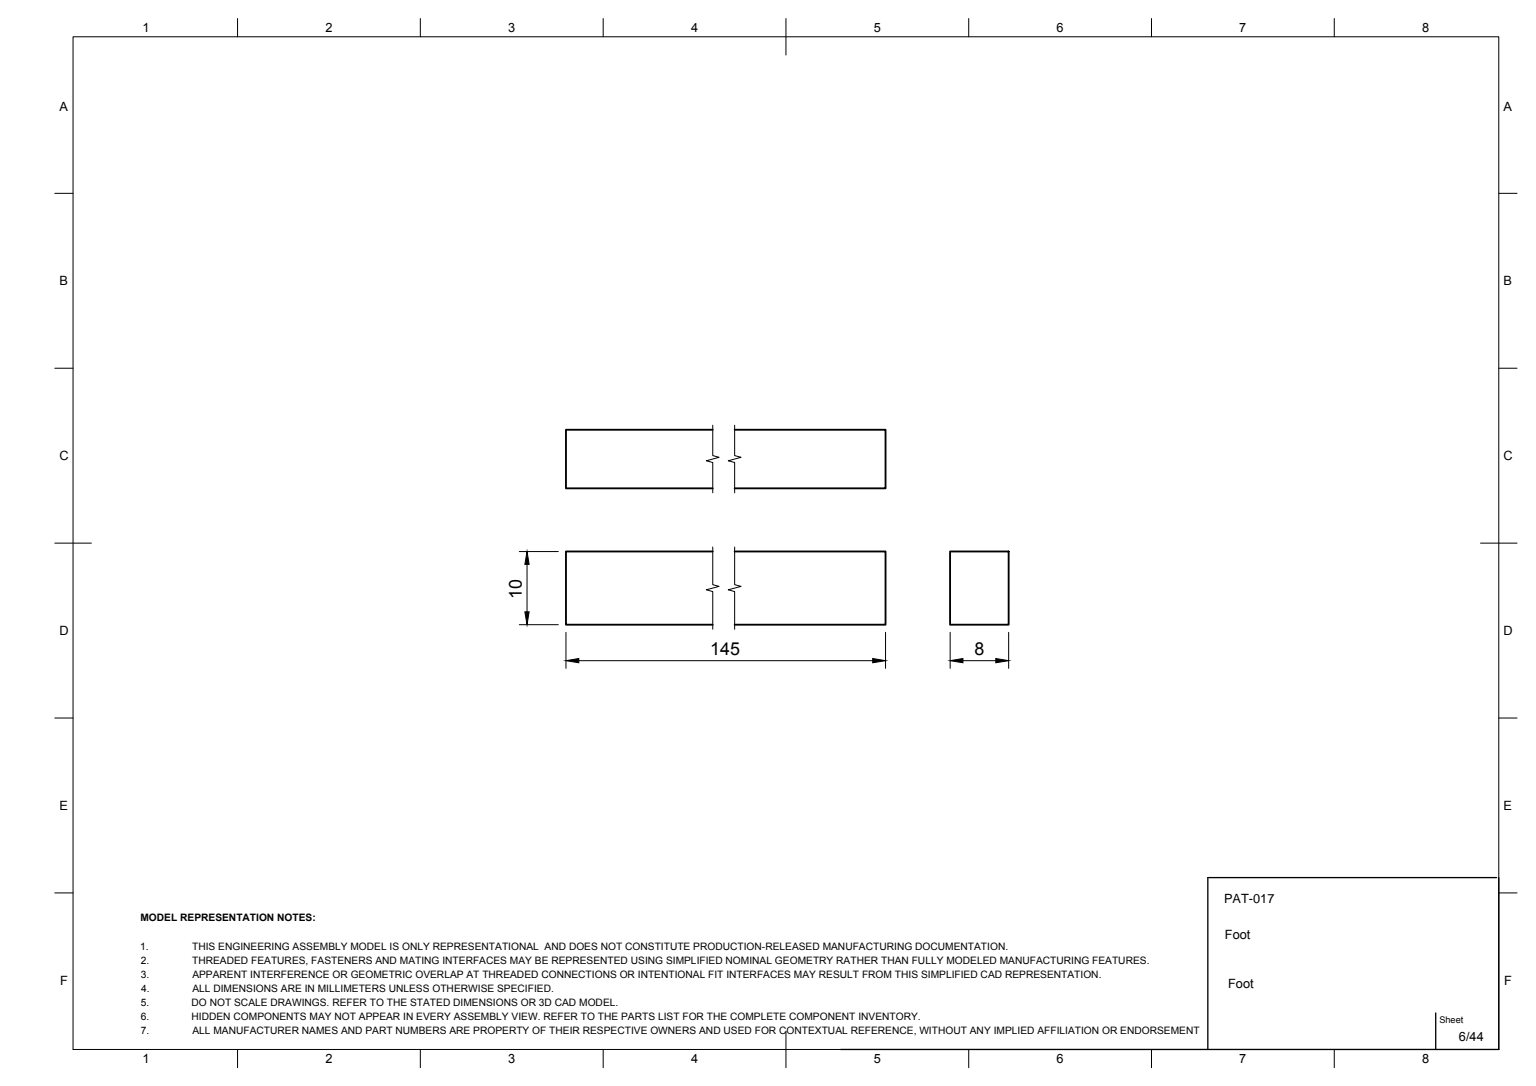
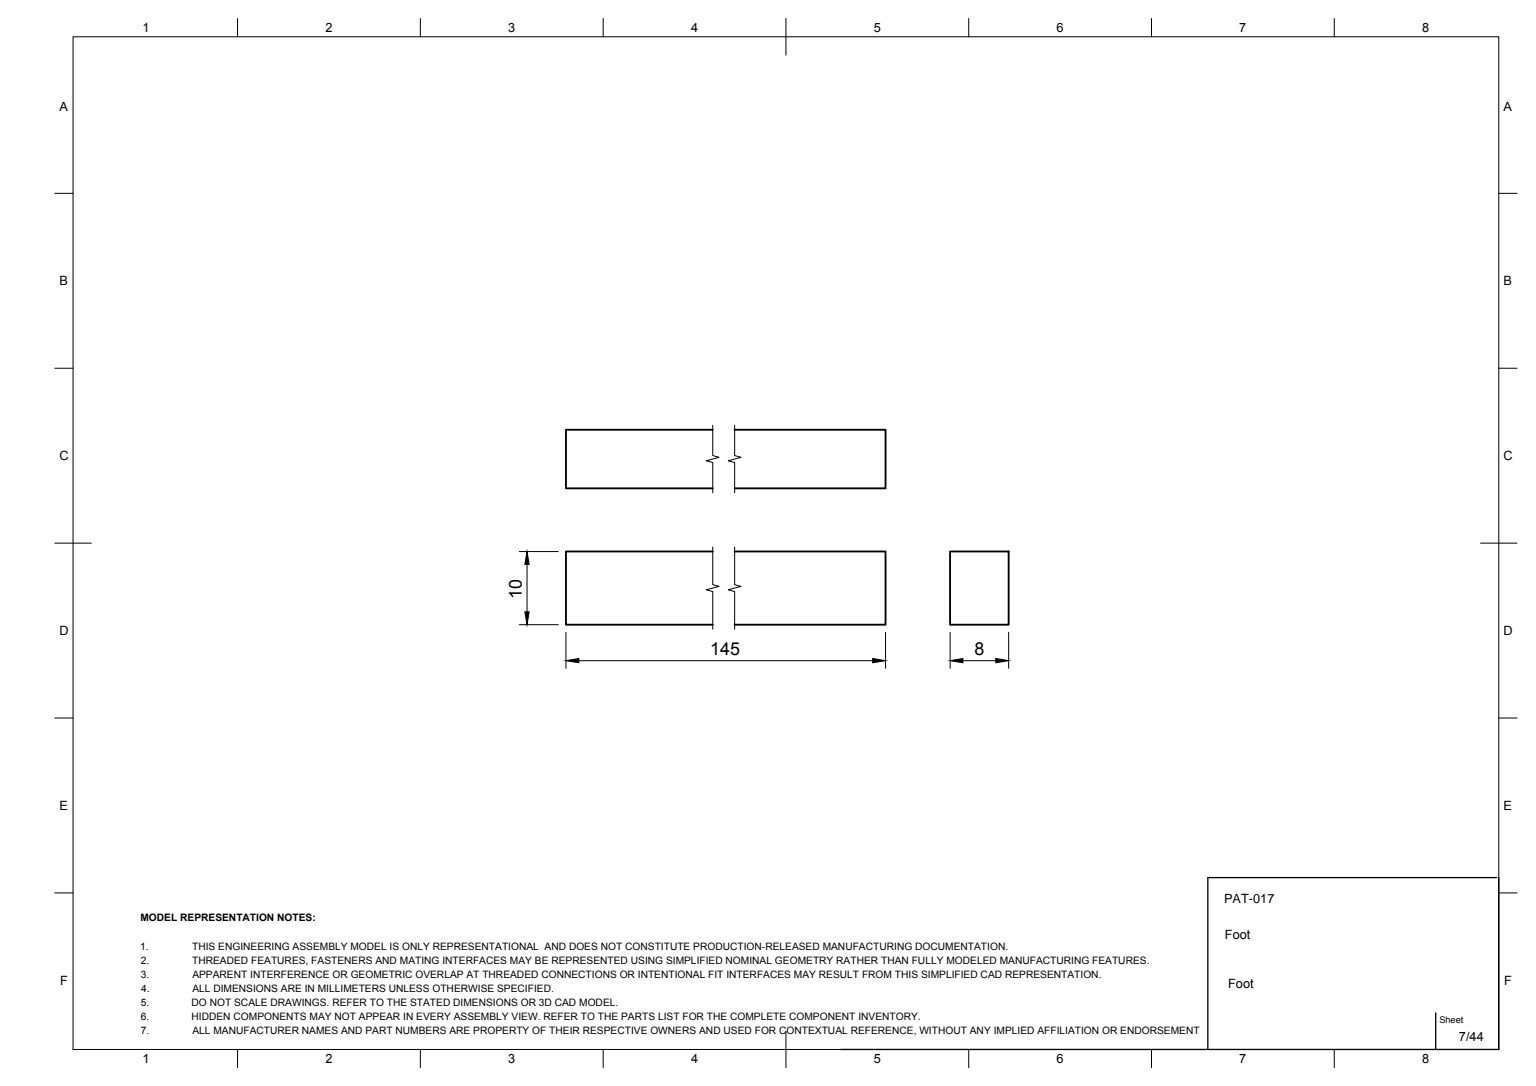
ISO-10303-21;
HEADER;
/* Generated by software containing ST-Developer
 * from STEP Tools, Inc. (www.steptools.com) 
 */

FILE_DESCRIPTION(
/* description */ ('Cam-and-follower valve demonstrator'),
/* implementation_level */ '2;1');

FILE_NAME(
/* name */ 'Foot.step',
/* time_stamp */ '2026-10-28T03:25:17-07:00',
/* author */ (''),
/* organization */ (''),
/* preprocessor_version */ 'ST-DEVELOPER v20.2',
/* originating_system */ 'Autodesk Translation Framework v15.17.0.0',
/* authorisation */ '');

FILE_SCHEMA (('AUTOMOTIVE_DESIGN { 1 0 10303 214 3 1 1 }'));
ENDSEC;

DATA;
#10=MECHANICAL_DESIGN_GEOMETRIC_PRESENTATION_REPRESENTATION('',(#413),#12896);
#341=SHAPE_REPRESENTATION_RELATIONSHIP('SRR','None',#13057,#377);
#377=ADVANCED_BREP_SHAPE_REPRESENTATION('',(#456),#12857);
#413=STYLED_ITEM('',(#13344),#456);
#456=MANIFOLD_SOLID_BREP('Body1',#6180);
#1112=FACE_OUTER_BOUND('',#1493,.T.);
#1113=FACE_OUTER_BOUND('',#1494,.T.);
#1114=FACE_OUTER_BOUND('',#1495,.T.);
#1115=FACE_OUTER_BOUND('',#1496,.T.);
#1116=FACE_OUTER_BOUND('',#1497,.T.);
#1117=FACE_OUTER_BOUND('',#1498,.T.);
#1493=EDGE_LOOP('',(#4179,#4180,#4181,#4182));
#1494=EDGE_LOOP('',(#4183,#4184,#4185,#4186));
#1495=EDGE_LOOP('',(#4187,#4188,#4189,#4190));
#1496=EDGE_LOOP('',(#4191,#4192,#4193,#4194));
#1497=EDGE_LOOP('',(#4195,#4196,#4197,#4198));
#1498=EDGE_LOOP('',(#4199,#4200,#4201,#4202));
#2025=LINE('',#9514,#2447);
#2026=LINE('',#9516,#2448);
#2027=LINE('',#9518,#2449);
#2028=LINE('',#9519,#2450);
#2029=LINE('',#9522,#2451);
#2030=LINE('',#9524,#2452);
#2031=LINE('',#9525,#2453);
#2032=LINE('',#9528,#2454);
#2033=LINE('',#9530,#2455);
#2034=LINE('',#9531,#2456);
#2035=LINE('',#9533,#2457);
#2036=LINE('',#9534,#2458);
#2447=VECTOR('',#7512,1.);
#2448=VECTOR('',#7513,1.);
#2449=VECTOR('',#7514,1.);
#2450=VECTOR('',#7515,1.);
#2451=VECTOR('',#7518,1.);
#2452=VECTOR('',#7519,1.);
#2453=VECTOR('',#7520,1.);
#2454=VECTOR('',#7523,1.);
#2455=VECTOR('',#7524,1.);
#2456=VECTOR('',#7525,1.);
#2457=VECTOR('',#7528,1.);
#2458=VECTOR('',#7529,1.);
#2867=VERTEX_POINT('',#9512);
#2868=VERTEX_POINT('',#9513);
#2869=VERTEX_POINT('',#9515);
#2870=VERTEX_POINT('',#9517);
#2871=VERTEX_POINT('',#9521);
#2872=VERTEX_POINT('',#9523);
#2873=VERTEX_POINT('',#9527);
#2874=VERTEX_POINT('',#9529);
#3386=EDGE_CURVE('',#2867,#2868,#2025,.T.);
#3387=EDGE_CURVE('',#2868,#2869,#2026,.T.);
#3388=EDGE_CURVE('',#2870,#2869,#2027,.T.);
#3389=EDGE_CURVE('',#2867,#2870,#2028,.T.);
#3390=EDGE_CURVE('',#2871,#2867,#2029,.T.);
#3391=EDGE_CURVE('',#2872,#2870,#2030,.T.);
#3392=EDGE_CURVE('',#2871,#2872,#2031,.T.);
#3393=EDGE_CURVE('',#2873,#2871,#2032,.T.);
#3394=EDGE_CURVE('',#2874,#2872,#2033,.T.);
#3395=EDGE_CURVE('',#2873,#2874,#2034,.T.);
#3396=EDGE_CURVE('',#2868,#2873,#2035,.T.);
#3397=EDGE_CURVE('',#2869,#2874,#2036,.T.);
#4179=ORIENTED_EDGE('',*,*,#3386,.T.);
#4180=ORIENTED_EDGE('',*,*,#3387,.T.);
#4181=ORIENTED_EDGE('',*,*,#3388,.F.);
#4182=ORIENTED_EDGE('',*,*,#3389,.F.);
#4183=ORIENTED_EDGE('',*,*,#3390,.T.);
#4184=ORIENTED_EDGE('',*,*,#3389,.T.);
#4185=ORIENTED_EDGE('',*,*,#3391,.F.);
#4186=ORIENTED_EDGE('',*,*,#3392,.F.);
#4187=ORIENTED_EDGE('',*,*,#3393,.T.);
#4188=ORIENTED_EDGE('',*,*,#3392,.T.);
#4189=ORIENTED_EDGE('',*,*,#3394,.F.);
#4190=ORIENTED_EDGE('',*,*,#3395,.F.);
#4191=ORIENTED_EDGE('',*,*,#3396,.T.);
#4192=ORIENTED_EDGE('',*,*,#3395,.T.);
#4193=ORIENTED_EDGE('',*,*,#3397,.F.);
#4194=ORIENTED_EDGE('',*,*,#3387,.F.);
#4195=ORIENTED_EDGE('',*,*,#3397,.T.);
#4196=ORIENTED_EDGE('',*,*,#3394,.T.);
#4197=ORIENTED_EDGE('',*,*,#3391,.T.);
#4198=ORIENTED_EDGE('',*,*,#3388,.T.);
#4199=ORIENTED_EDGE('',*,*,#3396,.F.);
#4200=ORIENTED_EDGE('',*,*,#3386,.F.);
#4201=ORIENTED_EDGE('',*,*,#3390,.F.);
#4202=ORIENTED_EDGE('',*,*,#3393,.F.);
#5608=PLANE('',#6655);
#5609=PLANE('',#6656);
#5610=PLANE('',#6657);
#5611=PLANE('',#6658);
#5612=PLANE('',#6659);
#5613=PLANE('',#6660);
#5828=ADVANCED_FACE('',(#1112),#5608,.T.);
#5829=ADVANCED_FACE('',(#1113),#5609,.T.);
#5830=ADVANCED_FACE('',(#1114),#5610,.T.);
#5831=ADVANCED_FACE('',(#1115),#5611,.T.);
#5832=ADVANCED_FACE('',(#1116),#5612,.T.);
#5833=ADVANCED_FACE('',(#1117),#5613,.F.);
#6180=CLOSED_SHELL('',(#5828,#5829,#5830,#5831,#5832,#5833));
#6654=AXIS2_PLACEMENT_3D('',#9510,#7508,#7509);
#6655=AXIS2_PLACEMENT_3D('',#9511,#7510,#7511);
#6656=AXIS2_PLACEMENT_3D('',#9520,#7516,#7517);
#6657=AXIS2_PLACEMENT_3D('',#9526,#7521,#7522);
#6658=AXIS2_PLACEMENT_3D('',#9532,#7526,#7527);
#6659=AXIS2_PLACEMENT_3D('',#9535,#7530,#7531);
#6660=AXIS2_PLACEMENT_3D('',#9536,#7532,#7533);
#7508=DIRECTION('axis',(0.,0.,1.));
#7509=DIRECTION('refdir',(1.,0.,0.));
#7510=DIRECTION('center_axis',(0.,1.,0.));
#7511=DIRECTION('ref_axis',(-1.,0.,0.));
#7512=DIRECTION('',(-1.,0.,0.));
#7513=DIRECTION('',(0.,0.,1.));
#7514=DIRECTION('',(-1.,0.,0.));
#7515=DIRECTION('',(0.,0.,1.));
#7516=DIRECTION('center_axis',(1.,0.,0.));
#7517=DIRECTION('ref_axis',(0.,1.,0.));
#7518=DIRECTION('',(0.,1.,0.));
#7519=DIRECTION('',(0.,1.,0.));
#7520=DIRECTION('',(0.,0.,1.));
#7521=DIRECTION('center_axis',(0.,-1.,0.));
#7522=DIRECTION('ref_axis',(1.,0.,0.));
#7523=DIRECTION('',(1.,0.,0.));
#7524=DIRECTION('',(1.,0.,0.));
#7525=DIRECTION('',(0.,0.,1.));
#7526=DIRECTION('center_axis',(-1.,0.,0.));
#7527=DIRECTION('ref_axis',(0.,-1.,0.));
#7528=DIRECTION('',(0.,-1.,0.));
#7529=DIRECTION('',(0.,-1.,0.));
#7530=DIRECTION('center_axis',(0.,0.,1.));
#7531=DIRECTION('ref_axis',(1.,0.,0.));
#7532=DIRECTION('center_axis',(0.,0.,1.));
#7533=DIRECTION('ref_axis',(1.,0.,0.));
#9510=CARTESIAN_POINT('',(0.,0.,0.));
#9511=CARTESIAN_POINT('Origin',(-5.,9.,-0.8));
#9512=CARTESIAN_POINT('',(-5.,9.,-0.8));
#9513=CARTESIAN_POINT('',(-6.,9.,-0.8));
#9514=CARTESIAN_POINT('',(-5.,9.,-0.8));
#9515=CARTESIAN_POINT('',(-6.,9.,0.));
#9516=CARTESIAN_POINT('',(-6.,9.,-0.8));
#9517=CARTESIAN_POINT('',(-5.,9.,0.));
#9518=CARTESIAN_POINT('',(-5.,9.,0.));
#9519=CARTESIAN_POINT('',(-5.,9.,-0.8));
#9520=CARTESIAN_POINT('Origin',(-5.,-5.5,-0.8));
#9521=CARTESIAN_POINT('',(-5.,-5.5,-0.8));
#9522=CARTESIAN_POINT('',(-5.,-5.5,-0.8));
#9523=CARTESIAN_POINT('',(-5.,-5.5,0.));
#9524=CARTESIAN_POINT('',(-5.,-5.5,0.));
#9525=CARTESIAN_POINT('',(-5.,-5.5,-0.8));
#9526=CARTESIAN_POINT('Origin',(-6.,-5.5,-0.8));
#9527=CARTESIAN_POINT('',(-6.,-5.5,-0.8));
#9528=CARTESIAN_POINT('',(-6.,-5.5,-0.8));
#9529=CARTESIAN_POINT('',(-6.,-5.5,0.));
#9530=CARTESIAN_POINT('',(-6.,-5.5,0.));
#9531=CARTESIAN_POINT('',(-6.,-5.5,-0.8));
#9532=CARTESIAN_POINT('Origin',(-6.,9.,-0.8));
#9533=CARTESIAN_POINT('',(-6.,9.,-0.8));
#9534=CARTESIAN_POINT('',(-6.,9.,0.));
#9535=CARTESIAN_POINT('Origin',(-5.5,1.75,0.));
#9536=CARTESIAN_POINT('Origin',(-5.5,1.75,-0.8));
#12814=UNCERTAINTY_MEASURE_WITH_UNIT(LENGTH_MEASURE(0.001),#12897,
'DISTANCE_ACCURACY_VALUE',
'Maximum model space distance between geometric entities at asserted c
onnectivities');
#12853=UNCERTAINTY_MEASURE_WITH_UNIT(LENGTH_MEASURE(0.001),#12897,
'DISTANCE_ACCURACY_VALUE',
'Maximum model space distance between geometric entities at asserted c
onnectivities');
#12857=(
GEOMETRIC_REPRESENTATION_CONTEXT(3)
GLOBAL_UNCERTAINTY_ASSIGNED_CONTEXT((#12814))
GLOBAL_UNIT_ASSIGNED_CONTEXT((#12897,#12899,#12900))
REPRESENTATION_CONTEXT('','3D')
);
#12896=(
GEOMETRIC_REPRESENTATION_CONTEXT(3)
GLOBAL_UNCERTAINTY_ASSIGNED_CONTEXT((#12853))
GLOBAL_UNIT_ASSIGNED_CONTEXT((#12897,#12899,#12900))
REPRESENTATION_CONTEXT('','3D')
);
#12897=(
LENGTH_UNIT()
NAMED_UNIT(*)
SI_UNIT(.CENTI.,.METRE.)
);
#12899=(
NAMED_UNIT(*)
PLANE_ANGLE_UNIT()
SI_UNIT($,.RADIAN.)
);
#12900=(
NAMED_UNIT(*)
SI_UNIT($,.STERADIAN.)
SOLID_ANGLE_UNIT()
);
#12904=SHAPE_DEFINITION_REPRESENTATION(#12946,#13057);
#12946=PRODUCT_DEFINITION_SHAPE('',$,#13100);
#13057=SHAPE_REPRESENTATION('',(#6654),#12857);
#13096=PRODUCT_DEFINITION_CONTEXT('part definition',#13224,'design');
#13100=PRODUCT_DEFINITION('Foot','Foot',#13142,#13096);
#13142=PRODUCT_DEFINITION_FORMATION('',$,#13229);
#13224=APPLICATION_CONTEXT(
'Core Data for Automotive Mechanical Design Process');
#13225=PRODUCT_CONTEXT('part definition',#13224,'mechanical');
#13229=PRODUCT('Foot','Foot','Foot',(#13225));
#13338=COLOUR_RGB('Off White',0.89,0.88,0.83);
#13339=FILL_AREA_STYLE_COLOUR('',#13338);
#13340=FILL_AREA_STYLE('',(#13339));
#13341=SURFACE_STYLE_FILL_AREA(#13340);
#13342=SURFACE_SIDE_STYLE('',(#13341));
#13343=SURFACE_STYLE_USAGE(.BOTH.,#13342);
#13344=PRESENTATION_STYLE_ASSIGNMENT((#13343));
ENDSEC;
END-ISO-10303-21;
